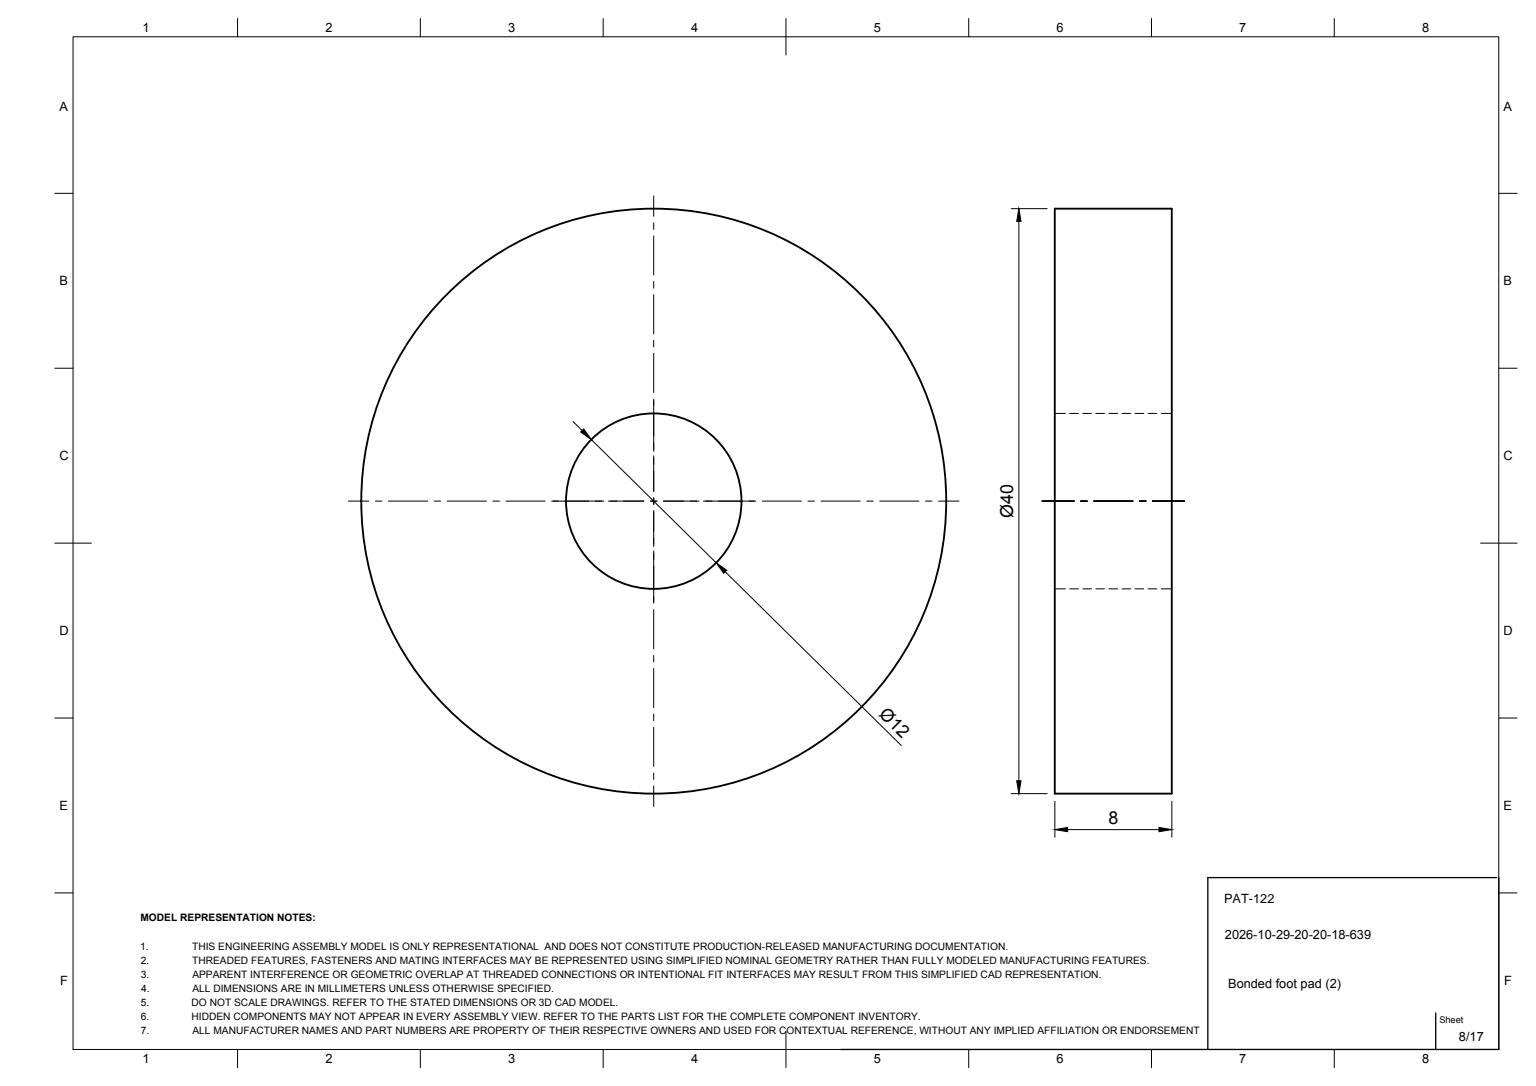
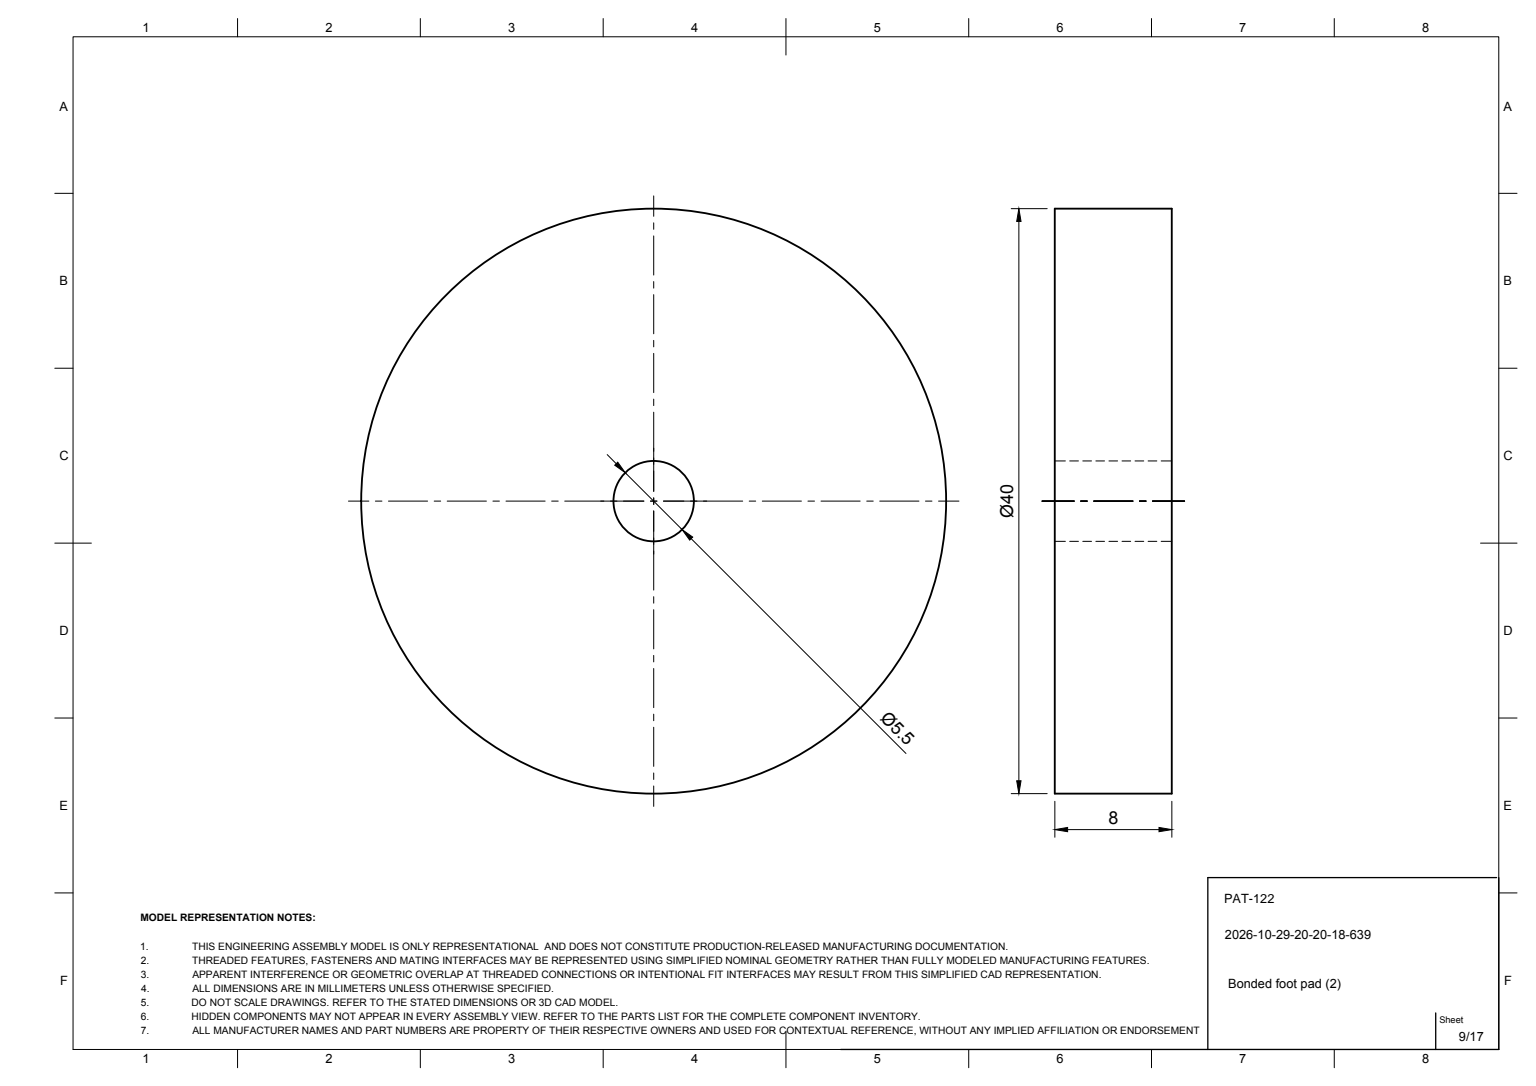
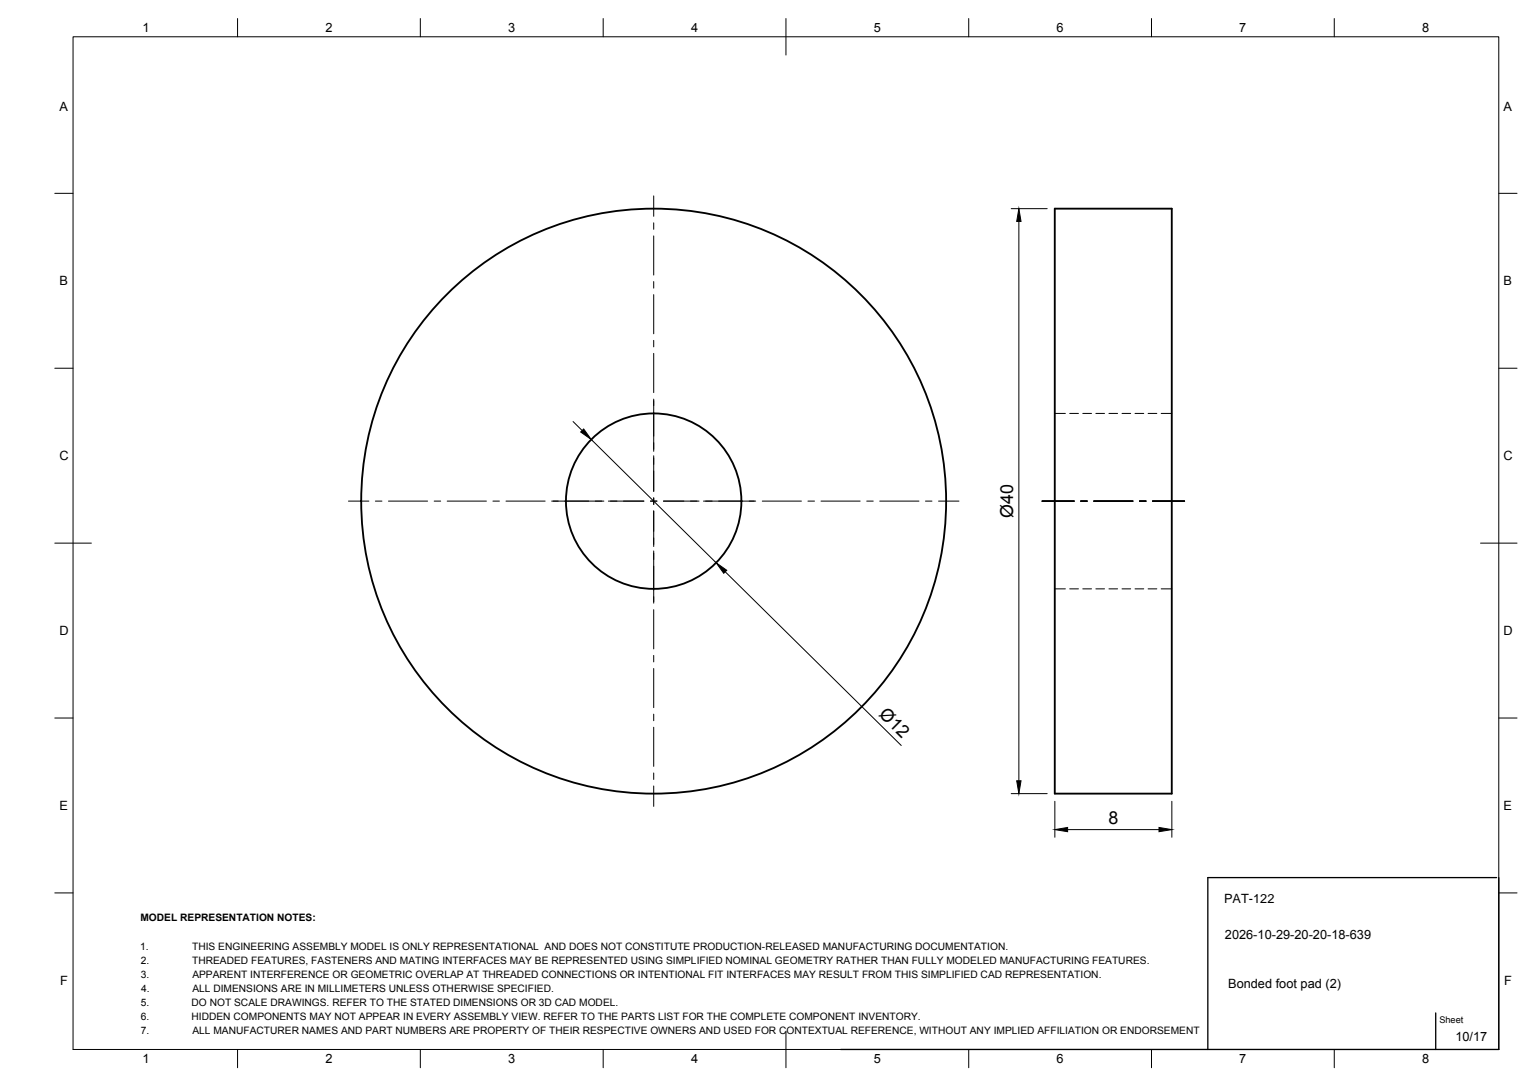
ISO-10303-21;
HEADER;
/* Generated by software containing ST-Developer
 * from STEP Tools, Inc. (www.steptools.com) 
 */

FILE_DESCRIPTION(
/* description */ ('PAT-122'),
/* implementation_level */ '2;1');

FILE_NAME(
/* name */ 'Bonded foot pad (2).step',
/* time_stamp */ '2026-10-29T20:20:12-07:00',
/* author */ (''),
/* organization */ (''),
/* preprocessor_version */ 'ST-DEVELOPER v20.2',
/* originating_system */ 'Autodesk Translation Framework v15.17.0.0',
/* authorisation */ '');

FILE_SCHEMA (('AUTOMOTIVE_DESIGN { 1 0 10303 214 3 1 1 }'));
ENDSEC;

DATA;
#10=MECHANICAL_DESIGN_GEOMETRIC_PRESENTATION_REPRESENTATION('',(#496),#10019);
#452=SHAPE_REPRESENTATION_RELATIONSHIP('SRR','None',#10173,#474);
#474=ADVANCED_BREP_SHAPE_REPRESENTATION('',(#518),#10002);
#496=STYLED_ITEM('',(#10341),#518);
#518=MANIFOLD_SOLID_BREP('Body1',#5618);
#541=FACE_BOUND('',#1150,.T.);
#542=FACE_BOUND('',#1152,.T.);
#619=PLANE('',#5935);
#620=PLANE('',#5936);
#845=FACE_OUTER_BOUND('',#1147,.T.);
#846=FACE_OUTER_BOUND('',#1148,.T.);
#847=FACE_OUTER_BOUND('',#1149,.T.);
#848=FACE_OUTER_BOUND('',#1151,.T.);
#1147=EDGE_LOOP('',(#3925,#3926,#3927,#3928));
#1148=EDGE_LOOP('',(#3929,#3930,#3931,#3932));
#1149=EDGE_LOOP('',(#3933));
#1150=EDGE_LOOP('',(#3934));
#1151=EDGE_LOOP('',(#3935));
#1152=EDGE_LOOP('',(#3936));
#1497=LINE('',#8139,#2041);
#1498=LINE('',#8145,#2042);
#2041=VECTOR('',#6534,0.600000000000001);
#2042=VECTOR('',#6541,2.);
#2595=CIRCLE('',#5930,0.600000000000001);
#2596=CIRCLE('',#5931,0.600000000000001);
#2597=CIRCLE('',#5933,2.);
#2598=CIRCLE('',#5934,2.);
#2725=VERTEX_POINT('',#8136);
#2726=VERTEX_POINT('',#8138);
#2727=VERTEX_POINT('',#8142);
#2728=VERTEX_POINT('',#8144);
#3197=EDGE_CURVE('',#2725,#2725,#2595,.T.);
#3198=EDGE_CURVE('',#2725,#2726,#1497,.T.);
#3199=EDGE_CURVE('',#2726,#2726,#2596,.T.);
#3200=EDGE_CURVE('',#2727,#2727,#2597,.T.);
#3201=EDGE_CURVE('',#2727,#2728,#1498,.T.);
#3202=EDGE_CURVE('',#2728,#2728,#2598,.T.);
#3925=ORIENTED_EDGE('',*,*,#3197,.F.);
#3926=ORIENTED_EDGE('',*,*,#3198,.T.);
#3927=ORIENTED_EDGE('',*,*,#3199,.T.);
#3928=ORIENTED_EDGE('',*,*,#3198,.F.);
#3929=ORIENTED_EDGE('',*,*,#3200,.F.);
#3930=ORIENTED_EDGE('',*,*,#3201,.T.);
#3931=ORIENTED_EDGE('',*,*,#3202,.T.);
#3932=ORIENTED_EDGE('',*,*,#3201,.F.);
#3933=ORIENTED_EDGE('',*,*,#3200,.T.);
#3934=ORIENTED_EDGE('',*,*,#3197,.T.);
#3935=ORIENTED_EDGE('',*,*,#3202,.F.);
#3936=ORIENTED_EDGE('',*,*,#3199,.F.);
#5271=CYLINDRICAL_SURFACE('',#5929,0.600000000000001);
#5272=CYLINDRICAL_SURFACE('',#5932,2.);
#5341=ADVANCED_FACE('',(#845),#5271,.F.);
#5342=ADVANCED_FACE('',(#846),#5272,.T.);
#5343=ADVANCED_FACE('',(#847,#541),#619,.T.);
#5344=ADVANCED_FACE('',(#848,#542),#620,.F.);
#5618=CLOSED_SHELL('',(#5341,#5342,#5343,#5344));
#5928=AXIS2_PLACEMENT_3D('',#8134,#6528,#6529);
#5929=AXIS2_PLACEMENT_3D('',#8135,#6530,#6531);
#5930=AXIS2_PLACEMENT_3D('',#8137,#6532,#6533);
#5931=AXIS2_PLACEMENT_3D('',#8140,#6535,#6536);
#5932=AXIS2_PLACEMENT_3D('',#8141,#6537,#6538);
#5933=AXIS2_PLACEMENT_3D('',#8143,#6539,#6540);
#5934=AXIS2_PLACEMENT_3D('',#8146,#6542,#6543);
#5935=AXIS2_PLACEMENT_3D('',#8147,#6544,#6545);
#5936=AXIS2_PLACEMENT_3D('',#8148,#6546,#6547);
#6528=DIRECTION('axis',(0.,0.,1.));
#6529=DIRECTION('refdir',(1.,0.,0.));
#6530=DIRECTION('center_axis',(0.,0.,1.));
#6531=DIRECTION('ref_axis',(1.,0.,0.));
#6532=DIRECTION('center_axis',(0.,0.,-1.));
#6533=DIRECTION('ref_axis',(1.,0.,0.));
#6534=DIRECTION('',(0.,0.,-1.));
#6535=DIRECTION('center_axis',(0.,0.,-1.));
#6536=DIRECTION('ref_axis',(1.,0.,0.));
#6537=DIRECTION('center_axis',(0.,0.,1.));
#6538=DIRECTION('ref_axis',(1.,0.,0.));
#6539=DIRECTION('center_axis',(0.,0.,1.));
#6540=DIRECTION('ref_axis',(1.,0.,0.));
#6541=DIRECTION('',(0.,0.,-1.));
#6542=DIRECTION('center_axis',(0.,0.,1.));
#6543=DIRECTION('ref_axis',(1.,0.,0.));
#6544=DIRECTION('center_axis',(0.,0.,1.));
#6545=DIRECTION('ref_axis',(1.,0.,0.));
#6546=DIRECTION('center_axis',(0.,0.,1.));
#6547=DIRECTION('ref_axis',(1.,0.,0.));
#8134=CARTESIAN_POINT('',(0.,0.,0.));
#8135=CARTESIAN_POINT('Origin',(19.,-19.,-1.6));
#8136=CARTESIAN_POINT('',(18.4,-19.,-0.8));
#8137=CARTESIAN_POINT('Origin',(19.,-19.,-0.8));
#8138=CARTESIAN_POINT('',(18.4,-19.,-1.6));
#8139=CARTESIAN_POINT('',(18.4,-19.,-1.6));
#8140=CARTESIAN_POINT('Origin',(19.,-19.,-1.6));
#8141=CARTESIAN_POINT('Origin',(19.,-19.,-1.6));
#8142=CARTESIAN_POINT('',(17.,-19.,-0.8));
#8143=CARTESIAN_POINT('Origin',(19.,-19.,-0.8));
#8144=CARTESIAN_POINT('',(17.,-19.,-1.6));
#8145=CARTESIAN_POINT('',(17.,-19.,-1.6));
#8146=CARTESIAN_POINT('Origin',(19.,-19.,-1.6));
#8147=CARTESIAN_POINT('Origin',(19.,-19.,-0.8));
#8148=CARTESIAN_POINT('Origin',(19.,-19.,-1.6));
#9978=UNCERTAINTY_MEASURE_WITH_UNIT(LENGTH_MEASURE(0.001),#10020,
'DISTANCE_ACCURACY_VALUE',
'Maximum model space distance between geometric entities at asserted c
onnectivities');
#9995=UNCERTAINTY_MEASURE_WITH_UNIT(LENGTH_MEASURE(0.001),#10020,
'DISTANCE_ACCURACY_VALUE',
'Maximum model space distance between geometric entities at asserted c
onnectivities');
#10002=(
GEOMETRIC_REPRESENTATION_CONTEXT(3)
GLOBAL_UNCERTAINTY_ASSIGNED_CONTEXT((#9978))
GLOBAL_UNIT_ASSIGNED_CONTEXT((#10020,#10022,#10023))
REPRESENTATION_CONTEXT('','3D')
);
#10019=(
GEOMETRIC_REPRESENTATION_CONTEXT(3)
GLOBAL_UNCERTAINTY_ASSIGNED_CONTEXT((#9995))
GLOBAL_UNIT_ASSIGNED_CONTEXT((#10020,#10022,#10023))
REPRESENTATION_CONTEXT('','3D')
);
#10020=(
LENGTH_UNIT()
NAMED_UNIT(*)
SI_UNIT(.CENTI.,.METRE.)
);
#10022=(
NAMED_UNIT(*)
PLANE_ANGLE_UNIT()
SI_UNIT($,.RADIAN.)
);
#10023=(
NAMED_UNIT(*)
SI_UNIT($,.STERADIAN.)
SOLID_ANGLE_UNIT()
);
#10030=SHAPE_DEFINITION_REPRESENTATION(#10053,#10173);
#10053=PRODUCT_DEFINITION_SHAPE('',$,#10197);
#10173=SHAPE_REPRESENTATION('',(#5928),#10002);
#10190=PRODUCT_DEFINITION_CONTEXT('part definition',#10261,'design');
#10197=PRODUCT_DEFINITION('Bonded foot pad (2)',
'Bonded foot pad (2)',#10220,#10190);
#10220=PRODUCT_DEFINITION_FORMATION('',$,#10269);
#10261=APPLICATION_CONTEXT(
'Core Data for Automotive Mechanical Design Process');
#10262=PRODUCT_CONTEXT('part definition',#10261,'mechanical');
#10269=PRODUCT('Bonded foot pad (2)','Bonded foot pad (2)',
'Bonded foot pad (2)',(#10262));
#10335=COLOUR_RGB('Sky Blue',0.24,0.69,0.87);
#10336=FILL_AREA_STYLE_COLOUR('',#10335);
#10337=FILL_AREA_STYLE('',(#10336));
#10338=SURFACE_STYLE_FILL_AREA(#10337);
#10339=SURFACE_SIDE_STYLE('',(#10338));
#10340=SURFACE_STYLE_USAGE(.BOTH.,#10339);
#10341=PRESENTATION_STYLE_ASSIGNMENT((#10340));
ENDSEC;
END-ISO-10303-21;
